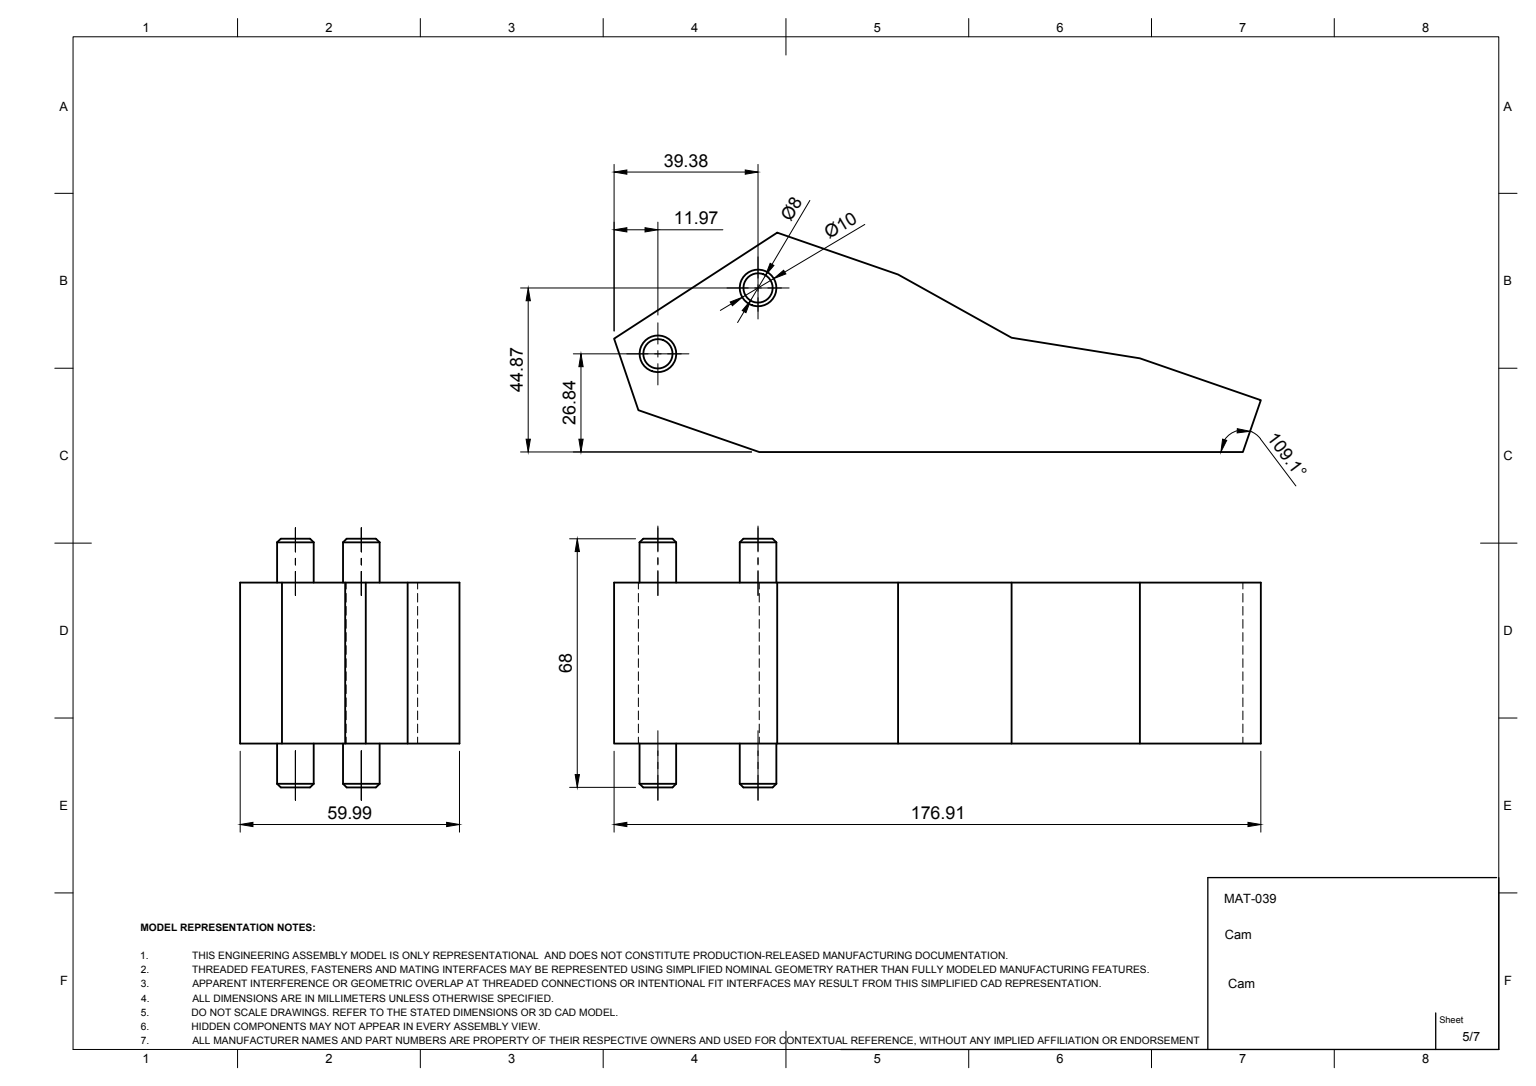
ISO-10303-21;
HEADER;
/* Generated by software containing ST-Developer
 * from STEP Tools, Inc. (www.steptools.com) 
 */

FILE_DESCRIPTION(
/* description */ ('STEP AP214'),
/* implementation_level */ '2;1');

FILE_NAME(
/* name */ 'Cam.step',
/* time_stamp */ '2026-11-14T21:46:24-08:00',
/* author */ (''),
/* organization */ (''),
/* preprocessor_version */ 'ST-DEVELOPER v20.2',
/* originating_system */ 'Autodesk Translation Framework v15.17.0.0',
/* authorisation */ '');

FILE_SCHEMA (('AUTOMOTIVE_DESIGN { 1 0 10303 214 3 1 1 }'));
ENDSEC;

DATA;
#10=MECHANICAL_DESIGN_GEOMETRIC_PRESENTATION_REPRESENTATION('',(#95),#7783);
#81=SHAPE_REPRESENTATION_RELATIONSHIP('SRR','None',#7826,#88);
#88=ADVANCED_BREP_SHAPE_REPRESENTATION('',(#102),#7782);
#95=STYLED_ITEM('',(#7871),#102);
#102=MANIFOLD_SOLID_BREP('Body1',#4170);
#108=CONICAL_SURFACE('',#4664,5.,0.785398163397445);
#109=CONICAL_SURFACE('',#4668,5.,0.785398163397445);
#110=CONICAL_SURFACE('',#4672,3.99999999999998,0.785398163397453);
#111=CONICAL_SURFACE('',#4675,3.99999999999998,0.785398163397453);
#155=FACE_BOUND('',#1601,.T.);
#156=FACE_BOUND('',#1602,.T.);
#157=FACE_BOUND('',#1604,.T.);
#158=FACE_BOUND('',#1605,.T.);
#274=PLANE('',#4686);
#275=PLANE('',#4687);
#276=PLANE('',#4688);
#277=PLANE('',#4689);
#278=PLANE('',#4690);
#279=PLANE('',#4691);
#280=PLANE('',#4692);
#281=PLANE('',#4693);
#282=PLANE('',#4694);
#283=PLANE('',#4695);
#284=PLANE('',#4696);
#285=PLANE('',#4697);
#286=PLANE('',#4698);
#287=PLANE('',#4699);
#288=PLANE('',#4700);
#613=LINE('',#7655,#972);
#614=LINE('',#7663,#973);
#615=LINE('',#7669,#974);
#616=LINE('',#7675,#975);
#617=LINE('',#7680,#976);
#618=LINE('',#7683,#977);
#619=LINE('',#7688,#978);
#620=LINE('',#7691,#979);
#621=LINE('',#7696,#980);
#622=LINE('',#7698,#981);
#623=LINE('',#7700,#982);
#624=LINE('',#7702,#983);
#625=LINE('',#7704,#984);
#626=LINE('',#7706,#985);
#627=LINE('',#7708,#986);
#628=LINE('',#7710,#987);
#629=LINE('',#7711,#988);
#630=LINE('',#7715,#989);
#631=LINE('',#7717,#990);
#632=LINE('',#7719,#991);
#633=LINE('',#7721,#992);
#634=LINE('',#7723,#993);
#635=LINE('',#7725,#994);
#636=LINE('',#7727,#995);
#637=LINE('',#7729,#996);
#638=LINE('',#7730,#997);
#639=LINE('',#7732,#998);
#640=LINE('',#7733,#999);
#641=LINE('',#7735,#1000);
#642=LINE('',#7737,#1001);
#643=LINE('',#7739,#1002);
#644=LINE('',#7741,#1003);
#645=LINE('',#7743,#1004);
#646=LINE('',#7745,#1005);
#647=LINE('',#7747,#1006);
#972=VECTOR('',#5872,5.);
#973=VECTOR('',#5881,5.);
#974=VECTOR('',#5888,3.99999999999998);
#975=VECTOR('',#5895,3.99999999999998);
#976=VECTOR('',#5902,5.);
#977=VECTOR('',#5905,5.);
#978=VECTOR('',#5912,5.);
#979=VECTOR('',#5915,5.);
#980=VECTOR('',#5920,1000.);
#981=VECTOR('',#5921,1000.);
#982=VECTOR('',#5922,1000.);
#983=VECTOR('',#5923,1000.);
#984=VECTOR('',#5924,1000.);
#985=VECTOR('',#5925,1000.);
#986=VECTOR('',#5926,1000.);
#987=VECTOR('',#5927,1000.);
#988=VECTOR('',#5928,1000.);
#989=VECTOR('',#5931,1000.);
#990=VECTOR('',#5932,1000.);
#991=VECTOR('',#5933,1000.);
#992=VECTOR('',#5934,1000.);
#993=VECTOR('',#5935,1000.);
#994=VECTOR('',#5936,1000.);
#995=VECTOR('',#5937,1000.);
#996=VECTOR('',#5938,1000.);
#997=VECTOR('',#5939,1000.);
#998=VECTOR('',#5942,1000.);
#999=VECTOR('',#5943,1000.);
#1000=VECTOR('',#5946,1000.);
#1001=VECTOR('',#5949,1000.);
#1002=VECTOR('',#5952,1000.);
#1003=VECTOR('',#5955,1000.);
#1004=VECTOR('',#5958,1000.);
#1005=VECTOR('',#5961,1000.);
#1006=VECTOR('',#5964,1000.);
#1082=CYLINDRICAL_SURFACE('',#4678,5.);
#1083=CYLINDRICAL_SURFACE('',#4680,5.);
#1084=CYLINDRICAL_SURFACE('',#4682,5.);
#1085=CYLINDRICAL_SURFACE('',#4684,5.);
#1306=FACE_OUTER_BOUND('',#1592,.T.);
#1307=FACE_OUTER_BOUND('',#1593,.T.);
#1308=FACE_OUTER_BOUND('',#1594,.T.);
#1309=FACE_OUTER_BOUND('',#1595,.T.);
#1310=FACE_OUTER_BOUND('',#1596,.T.);
#1311=FACE_OUTER_BOUND('',#1597,.T.);
#1312=FACE_OUTER_BOUND('',#1598,.T.);
#1313=FACE_OUTER_BOUND('',#1599,.T.);
#1314=FACE_OUTER_BOUND('',#1600,.T.);
#1315=FACE_OUTER_BOUND('',#1603,.T.);
#1316=FACE_OUTER_BOUND('',#1606,.T.);
#1317=FACE_OUTER_BOUND('',#1607,.T.);
#1318=FACE_OUTER_BOUND('',#1608,.T.);
#1319=FACE_OUTER_BOUND('',#1609,.T.);
#1320=FACE_OUTER_BOUND('',#1610,.T.);
#1321=FACE_OUTER_BOUND('',#1611,.T.);
#1322=FACE_OUTER_BOUND('',#1612,.T.);
#1323=FACE_OUTER_BOUND('',#1613,.T.);
#1324=FACE_OUTER_BOUND('',#1614,.T.);
#1325=FACE_OUTER_BOUND('',#1615,.T.);
#1326=FACE_OUTER_BOUND('',#1616,.T.);
#1327=FACE_OUTER_BOUND('',#1617,.T.);
#1328=FACE_OUTER_BOUND('',#1618,.T.);
#1592=EDGE_LOOP('',(#3804,#3805,#3806,#3807,#3808));
#1593=EDGE_LOOP('',(#3809,#3810,#3811,#3812,#3813));
#1594=EDGE_LOOP('',(#3814,#3815,#3816,#3817));
#1595=EDGE_LOOP('',(#3818,#3819,#3820,#3821));
#1596=EDGE_LOOP('',(#3822,#3823,#3824,#3825));
#1597=EDGE_LOOP('',(#3826,#3827,#3828,#3829,#3830));
#1598=EDGE_LOOP('',(#3831,#3832,#3833,#3834));
#1599=EDGE_LOOP('',(#3835,#3836,#3837,#3838,#3839));
#1600=EDGE_LOOP('',(#3840,#3841,#3842,#3843,#3844,#3845,#3846,#3847,#3848));
#1601=EDGE_LOOP('',(#3849));
#1602=EDGE_LOOP('',(#3850));
#1603=EDGE_LOOP('',(#3851,#3852,#3853,#3854,#3855,#3856,#3857,#3858,#3859));
#1604=EDGE_LOOP('',(#3860));
#1605=EDGE_LOOP('',(#3861));
#1606=EDGE_LOOP('',(#3862,#3863,#3864,#3865));
#1607=EDGE_LOOP('',(#3866,#3867,#3868,#3869));
#1608=EDGE_LOOP('',(#3870,#3871,#3872,#3873));
#1609=EDGE_LOOP('',(#3874,#3875,#3876,#3877));
#1610=EDGE_LOOP('',(#3878,#3879,#3880,#3881));
#1611=EDGE_LOOP('',(#3882,#3883,#3884,#3885));
#1612=EDGE_LOOP('',(#3886,#3887,#3888,#3889));
#1613=EDGE_LOOP('',(#3890,#3891,#3892,#3893));
#1614=EDGE_LOOP('',(#3894,#3895,#3896,#3897));
#1615=EDGE_LOOP('',(#3898));
#1616=EDGE_LOOP('',(#3899));
#1617=EDGE_LOOP('',(#3900));
#1618=EDGE_LOOP('',(#3901));
#1808=CIRCLE('',#4665,5.);
#1809=CIRCLE('',#4666,5.);
#1810=CIRCLE('',#4667,3.99999999999999);
#1811=CIRCLE('',#4669,5.);
#1812=CIRCLE('',#4670,5.);
#1813=CIRCLE('',#4671,3.99999999999999);
#1814=CIRCLE('',#4673,5.);
#1815=CIRCLE('',#4674,3.99999999999998);
#1816=CIRCLE('',#4676,5.);
#1817=CIRCLE('',#4677,3.99999999999998);
#1818=CIRCLE('',#4679,5.);
#1819=CIRCLE('',#4681,5.);
#1820=CIRCLE('',#4683,5.);
#1821=CIRCLE('',#4685,5.);
#2154=VERTEX_POINT('',#7650);
#2155=VERTEX_POINT('',#7651);
#2156=VERTEX_POINT('',#7654);
#2157=VERTEX_POINT('',#7658);
#2158=VERTEX_POINT('',#7659);
#2159=VERTEX_POINT('',#7662);
#2160=VERTEX_POINT('',#7666);
#2161=VERTEX_POINT('',#7668);
#2162=VERTEX_POINT('',#7672);
#2163=VERTEX_POINT('',#7674);
#2164=VERTEX_POINT('',#7678);
#2165=VERTEX_POINT('',#7682);
#2166=VERTEX_POINT('',#7686);
#2167=VERTEX_POINT('',#7690);
#2168=VERTEX_POINT('',#7694);
#2169=VERTEX_POINT('',#7695);
#2170=VERTEX_POINT('',#7697);
#2171=VERTEX_POINT('',#7699);
#2172=VERTEX_POINT('',#7701);
#2173=VERTEX_POINT('',#7703);
#2174=VERTEX_POINT('',#7705);
#2175=VERTEX_POINT('',#7707);
#2176=VERTEX_POINT('',#7709);
#2177=VERTEX_POINT('',#7713);
#2178=VERTEX_POINT('',#7714);
#2179=VERTEX_POINT('',#7716);
#2180=VERTEX_POINT('',#7718);
#2181=VERTEX_POINT('',#7720);
#2182=VERTEX_POINT('',#7722);
#2183=VERTEX_POINT('',#7724);
#2184=VERTEX_POINT('',#7726);
#2185=VERTEX_POINT('',#7728);
#2709=EDGE_CURVE('',#2154,#2155,#1808,.T.);
#2710=EDGE_CURVE('',#2155,#2154,#1809,.T.);
#2711=EDGE_CURVE('',#2155,#2156,#613,.T.);
#2712=EDGE_CURVE('',#2156,#2156,#1810,.T.);
#2713=EDGE_CURVE('',#2157,#2158,#1811,.T.);
#2714=EDGE_CURVE('',#2158,#2157,#1812,.T.);
#2715=EDGE_CURVE('',#2158,#2159,#614,.T.);
#2716=EDGE_CURVE('',#2159,#2159,#1813,.T.);
#2717=EDGE_CURVE('',#2160,#2160,#1814,.T.);
#2718=EDGE_CURVE('',#2160,#2161,#615,.T.);
#2719=EDGE_CURVE('',#2161,#2161,#1815,.T.);
#2720=EDGE_CURVE('',#2162,#2162,#1816,.T.);
#2721=EDGE_CURVE('',#2162,#2163,#616,.T.);
#2722=EDGE_CURVE('',#2163,#2163,#1817,.T.);
#2723=EDGE_CURVE('',#2164,#2164,#1818,.T.);
#2724=EDGE_CURVE('',#2164,#2162,#617,.T.);
#2725=EDGE_CURVE('',#2157,#2165,#618,.T.);
#2726=EDGE_CURVE('',#2165,#2165,#1819,.T.);
#2727=EDGE_CURVE('',#2166,#2166,#1820,.T.);
#2728=EDGE_CURVE('',#2166,#2160,#619,.T.);
#2729=EDGE_CURVE('',#2154,#2167,#620,.T.);
#2730=EDGE_CURVE('',#2167,#2167,#1821,.T.);
#2731=EDGE_CURVE('',#2168,#2169,#621,.T.);
#2732=EDGE_CURVE('',#2169,#2170,#622,.T.);
#2733=EDGE_CURVE('',#2170,#2171,#623,.T.);
#2734=EDGE_CURVE('',#2171,#2172,#624,.T.);
#2735=EDGE_CURVE('',#2172,#2173,#625,.T.);
#2736=EDGE_CURVE('',#2173,#2174,#626,.T.);
#2737=EDGE_CURVE('',#2174,#2175,#627,.T.);
#2738=EDGE_CURVE('',#2175,#2176,#628,.T.);
#2739=EDGE_CURVE('',#2176,#2168,#629,.T.);
#2740=EDGE_CURVE('',#2177,#2178,#630,.T.);
#2741=EDGE_CURVE('',#2179,#2177,#631,.T.);
#2742=EDGE_CURVE('',#2180,#2179,#632,.T.);
#2743=EDGE_CURVE('',#2181,#2180,#633,.T.);
#2744=EDGE_CURVE('',#2182,#2181,#634,.T.);
#2745=EDGE_CURVE('',#2183,#2182,#635,.T.);
#2746=EDGE_CURVE('',#2184,#2183,#636,.T.);
#2747=EDGE_CURVE('',#2185,#2184,#637,.T.);
#2748=EDGE_CURVE('',#2178,#2185,#638,.T.);
#2749=EDGE_CURVE('',#2169,#2178,#639,.T.);
#2750=EDGE_CURVE('',#2168,#2177,#640,.T.);
#2751=EDGE_CURVE('',#2170,#2185,#641,.T.);
#2752=EDGE_CURVE('',#2171,#2184,#642,.T.);
#2753=EDGE_CURVE('',#2172,#2183,#643,.T.);
#2754=EDGE_CURVE('',#2173,#2182,#644,.T.);
#2755=EDGE_CURVE('',#2174,#2181,#645,.T.);
#2756=EDGE_CURVE('',#2175,#2180,#646,.T.);
#2757=EDGE_CURVE('',#2176,#2179,#647,.T.);
#3804=ORIENTED_EDGE('',*,*,#2709,.F.);
#3805=ORIENTED_EDGE('',*,*,#2710,.F.);
#3806=ORIENTED_EDGE('',*,*,#2711,.T.);
#3807=ORIENTED_EDGE('',*,*,#2712,.F.);
#3808=ORIENTED_EDGE('',*,*,#2711,.F.);
#3809=ORIENTED_EDGE('',*,*,#2713,.F.);
#3810=ORIENTED_EDGE('',*,*,#2714,.F.);
#3811=ORIENTED_EDGE('',*,*,#2715,.T.);
#3812=ORIENTED_EDGE('',*,*,#2716,.F.);
#3813=ORIENTED_EDGE('',*,*,#2715,.F.);
#3814=ORIENTED_EDGE('',*,*,#2717,.F.);
#3815=ORIENTED_EDGE('',*,*,#2718,.T.);
#3816=ORIENTED_EDGE('',*,*,#2719,.F.);
#3817=ORIENTED_EDGE('',*,*,#2718,.F.);
#3818=ORIENTED_EDGE('',*,*,#2720,.F.);
#3819=ORIENTED_EDGE('',*,*,#2721,.T.);
#3820=ORIENTED_EDGE('',*,*,#2722,.F.);
#3821=ORIENTED_EDGE('',*,*,#2721,.F.);
#3822=ORIENTED_EDGE('',*,*,#2723,.T.);
#3823=ORIENTED_EDGE('',*,*,#2724,.T.);
#3824=ORIENTED_EDGE('',*,*,#2720,.T.);
#3825=ORIENTED_EDGE('',*,*,#2724,.F.);
#3826=ORIENTED_EDGE('',*,*,#2713,.T.);
#3827=ORIENTED_EDGE('',*,*,#2714,.T.);
#3828=ORIENTED_EDGE('',*,*,#2725,.T.);
#3829=ORIENTED_EDGE('',*,*,#2726,.T.);
#3830=ORIENTED_EDGE('',*,*,#2725,.F.);
#3831=ORIENTED_EDGE('',*,*,#2727,.T.);
#3832=ORIENTED_EDGE('',*,*,#2728,.T.);
#3833=ORIENTED_EDGE('',*,*,#2717,.T.);
#3834=ORIENTED_EDGE('',*,*,#2728,.F.);
#3835=ORIENTED_EDGE('',*,*,#2709,.T.);
#3836=ORIENTED_EDGE('',*,*,#2710,.T.);
#3837=ORIENTED_EDGE('',*,*,#2729,.T.);
#3838=ORIENTED_EDGE('',*,*,#2730,.T.);
#3839=ORIENTED_EDGE('',*,*,#2729,.F.);
#3840=ORIENTED_EDGE('',*,*,#2731,.T.);
#3841=ORIENTED_EDGE('',*,*,#2732,.T.);
#3842=ORIENTED_EDGE('',*,*,#2733,.T.);
#3843=ORIENTED_EDGE('',*,*,#2734,.T.);
#3844=ORIENTED_EDGE('',*,*,#2735,.T.);
#3845=ORIENTED_EDGE('',*,*,#2736,.T.);
#3846=ORIENTED_EDGE('',*,*,#2737,.T.);
#3847=ORIENTED_EDGE('',*,*,#2738,.T.);
#3848=ORIENTED_EDGE('',*,*,#2739,.T.);
#3849=ORIENTED_EDGE('',*,*,#2727,.F.);
#3850=ORIENTED_EDGE('',*,*,#2723,.F.);
#3851=ORIENTED_EDGE('',*,*,#2740,.F.);
#3852=ORIENTED_EDGE('',*,*,#2741,.F.);
#3853=ORIENTED_EDGE('',*,*,#2742,.F.);
#3854=ORIENTED_EDGE('',*,*,#2743,.F.);
#3855=ORIENTED_EDGE('',*,*,#2744,.F.);
#3856=ORIENTED_EDGE('',*,*,#2745,.F.);
#3857=ORIENTED_EDGE('',*,*,#2746,.F.);
#3858=ORIENTED_EDGE('',*,*,#2747,.F.);
#3859=ORIENTED_EDGE('',*,*,#2748,.F.);
#3860=ORIENTED_EDGE('',*,*,#2730,.F.);
#3861=ORIENTED_EDGE('',*,*,#2726,.F.);
#3862=ORIENTED_EDGE('',*,*,#2740,.T.);
#3863=ORIENTED_EDGE('',*,*,#2749,.F.);
#3864=ORIENTED_EDGE('',*,*,#2731,.F.);
#3865=ORIENTED_EDGE('',*,*,#2750,.T.);
#3866=ORIENTED_EDGE('',*,*,#2748,.T.);
#3867=ORIENTED_EDGE('',*,*,#2751,.F.);
#3868=ORIENTED_EDGE('',*,*,#2732,.F.);
#3869=ORIENTED_EDGE('',*,*,#2749,.T.);
#3870=ORIENTED_EDGE('',*,*,#2747,.T.);
#3871=ORIENTED_EDGE('',*,*,#2752,.F.);
#3872=ORIENTED_EDGE('',*,*,#2733,.F.);
#3873=ORIENTED_EDGE('',*,*,#2751,.T.);
#3874=ORIENTED_EDGE('',*,*,#2746,.T.);
#3875=ORIENTED_EDGE('',*,*,#2753,.F.);
#3876=ORIENTED_EDGE('',*,*,#2734,.F.);
#3877=ORIENTED_EDGE('',*,*,#2752,.T.);
#3878=ORIENTED_EDGE('',*,*,#2745,.T.);
#3879=ORIENTED_EDGE('',*,*,#2754,.F.);
#3880=ORIENTED_EDGE('',*,*,#2735,.F.);
#3881=ORIENTED_EDGE('',*,*,#2753,.T.);
#3882=ORIENTED_EDGE('',*,*,#2744,.T.);
#3883=ORIENTED_EDGE('',*,*,#2755,.F.);
#3884=ORIENTED_EDGE('',*,*,#2736,.F.);
#3885=ORIENTED_EDGE('',*,*,#2754,.T.);
#3886=ORIENTED_EDGE('',*,*,#2743,.T.);
#3887=ORIENTED_EDGE('',*,*,#2756,.F.);
#3888=ORIENTED_EDGE('',*,*,#2737,.F.);
#3889=ORIENTED_EDGE('',*,*,#2755,.T.);
#3890=ORIENTED_EDGE('',*,*,#2742,.T.);
#3891=ORIENTED_EDGE('',*,*,#2757,.F.);
#3892=ORIENTED_EDGE('',*,*,#2738,.F.);
#3893=ORIENTED_EDGE('',*,*,#2756,.T.);
#3894=ORIENTED_EDGE('',*,*,#2741,.T.);
#3895=ORIENTED_EDGE('',*,*,#2750,.F.);
#3896=ORIENTED_EDGE('',*,*,#2739,.F.);
#3897=ORIENTED_EDGE('',*,*,#2757,.T.);
#3898=ORIENTED_EDGE('',*,*,#2712,.T.);
#3899=ORIENTED_EDGE('',*,*,#2719,.T.);
#3900=ORIENTED_EDGE('',*,*,#2716,.T.);
#3901=ORIENTED_EDGE('',*,*,#2722,.T.);
#4141=ADVANCED_FACE('',(#1306),#108,.T.);
#4142=ADVANCED_FACE('',(#1307),#109,.T.);
#4143=ADVANCED_FACE('',(#1308),#110,.T.);
#4144=ADVANCED_FACE('',(#1309),#111,.T.);
#4145=ADVANCED_FACE('',(#1310),#1082,.T.);
#4146=ADVANCED_FACE('',(#1311),#1083,.T.);
#4147=ADVANCED_FACE('',(#1312),#1084,.T.);
#4148=ADVANCED_FACE('',(#1313),#1085,.T.);
#4149=ADVANCED_FACE('',(#1314,#155,#156),#274,.T.);
#4150=ADVANCED_FACE('',(#1315,#157,#158),#275,.F.);
#4151=ADVANCED_FACE('',(#1316),#276,.F.);
#4152=ADVANCED_FACE('',(#1317),#277,.F.);
#4153=ADVANCED_FACE('',(#1318),#278,.F.);
#4154=ADVANCED_FACE('',(#1319),#279,.F.);
#4155=ADVANCED_FACE('',(#1320),#280,.F.);
#4156=ADVANCED_FACE('',(#1321),#281,.F.);
#4157=ADVANCED_FACE('',(#1322),#282,.F.);
#4158=ADVANCED_FACE('',(#1323),#283,.F.);
#4159=ADVANCED_FACE('',(#1324),#284,.F.);
#4160=ADVANCED_FACE('',(#1325),#285,.F.);
#4161=ADVANCED_FACE('',(#1326),#286,.T.);
#4162=ADVANCED_FACE('',(#1327),#287,.F.);
#4163=ADVANCED_FACE('',(#1328),#288,.T.);
#4170=CLOSED_SHELL('',(#4141,#4142,#4143,#4144,#4145,#4146,#4147,#4148,
#4149,#4150,#4151,#4152,#4153,#4154,#4155,#4156,#4157,#4158,#4159,#4160,
#4161,#4162,#4163));
#4663=AXIS2_PLACEMENT_3D('',#7648,#5864,#5865);
#4664=AXIS2_PLACEMENT_3D('',#7649,#5866,#5867);
#4665=AXIS2_PLACEMENT_3D('',#7652,#5868,#5869);
#4666=AXIS2_PLACEMENT_3D('',#7653,#5870,#5871);
#4667=AXIS2_PLACEMENT_3D('',#7656,#5873,#5874);
#4668=AXIS2_PLACEMENT_3D('',#7657,#5875,#5876);
#4669=AXIS2_PLACEMENT_3D('',#7660,#5877,#5878);
#4670=AXIS2_PLACEMENT_3D('',#7661,#5879,#5880);
#4671=AXIS2_PLACEMENT_3D('',#7664,#5882,#5883);
#4672=AXIS2_PLACEMENT_3D('',#7665,#5884,#5885);
#4673=AXIS2_PLACEMENT_3D('',#7667,#5886,#5887);
#4674=AXIS2_PLACEMENT_3D('',#7670,#5889,#5890);
#4675=AXIS2_PLACEMENT_3D('',#7671,#5891,#5892);
#4676=AXIS2_PLACEMENT_3D('',#7673,#5893,#5894);
#4677=AXIS2_PLACEMENT_3D('',#7676,#5896,#5897);
#4678=AXIS2_PLACEMENT_3D('',#7677,#5898,#5899);
#4679=AXIS2_PLACEMENT_3D('',#7679,#5900,#5901);
#4680=AXIS2_PLACEMENT_3D('',#7681,#5903,#5904);
#4681=AXIS2_PLACEMENT_3D('',#7684,#5906,#5907);
#4682=AXIS2_PLACEMENT_3D('',#7685,#5908,#5909);
#4683=AXIS2_PLACEMENT_3D('',#7687,#5910,#5911);
#4684=AXIS2_PLACEMENT_3D('',#7689,#5913,#5914);
#4685=AXIS2_PLACEMENT_3D('',#7692,#5916,#5917);
#4686=AXIS2_PLACEMENT_3D('',#7693,#5918,#5919);
#4687=AXIS2_PLACEMENT_3D('',#7712,#5929,#5930);
#4688=AXIS2_PLACEMENT_3D('',#7731,#5940,#5941);
#4689=AXIS2_PLACEMENT_3D('',#7734,#5944,#5945);
#4690=AXIS2_PLACEMENT_3D('',#7736,#5947,#5948);
#4691=AXIS2_PLACEMENT_3D('',#7738,#5950,#5951);
#4692=AXIS2_PLACEMENT_3D('',#7740,#5953,#5954);
#4693=AXIS2_PLACEMENT_3D('',#7742,#5956,#5957);
#4694=AXIS2_PLACEMENT_3D('',#7744,#5959,#5960);
#4695=AXIS2_PLACEMENT_3D('',#7746,#5962,#5963);
#4696=AXIS2_PLACEMENT_3D('',#7748,#5965,#5966);
#4697=AXIS2_PLACEMENT_3D('',#7749,#5967,#5968);
#4698=AXIS2_PLACEMENT_3D('',#7750,#5969,#5970);
#4699=AXIS2_PLACEMENT_3D('',#7751,#5971,#5972);
#4700=AXIS2_PLACEMENT_3D('',#7752,#5973,#5974);
#5864=DIRECTION('axis',(0.,0.,1.));
#5865=DIRECTION('refdir',(1.,0.,0.));
#5866=DIRECTION('center_axis',(0.,0.,1.));
#5867=DIRECTION('ref_axis',(1.,0.,0.));
#5868=DIRECTION('center_axis',(0.,0.,1.));
#5869=DIRECTION('ref_axis',(1.,0.,0.));
#5870=DIRECTION('center_axis',(0.,0.,1.));
#5871=DIRECTION('ref_axis',(1.,0.,0.));
#5872=DIRECTION('',(0.707106781186545,8.6595605623549E-17,-0.70710678118655));
#5873=DIRECTION('center_axis',(0.,0.,-1.));
#5874=DIRECTION('ref_axis',(1.,0.,0.));
#5875=DIRECTION('center_axis',(0.,0.,1.));
#5876=DIRECTION('ref_axis',(1.,0.,0.));
#5877=DIRECTION('center_axis',(0.,0.,1.));
#5878=DIRECTION('ref_axis',(1.,0.,0.));
#5879=DIRECTION('center_axis',(0.,0.,1.));
#5880=DIRECTION('ref_axis',(1.,0.,0.));
#5881=DIRECTION('',(0.707106781186545,8.6595605623549E-17,-0.70710678118655));
#5882=DIRECTION('center_axis',(0.,0.,-1.));
#5883=DIRECTION('ref_axis',(1.,0.,0.));
#5884=DIRECTION('center_axis',(0.,0.,-1.));
#5885=DIRECTION('ref_axis',(-1.,0.,0.));
#5886=DIRECTION('center_axis',(0.,0.,-1.));
#5887=DIRECTION('ref_axis',(1.,0.,0.));
#5888=DIRECTION('',(-0.707106781186551,8.65956056235498E-17,0.707106781186544));
#5889=DIRECTION('center_axis',(0.,0.,1.));
#5890=DIRECTION('ref_axis',(1.,0.,0.));
#5891=DIRECTION('center_axis',(0.,0.,-1.));
#5892=DIRECTION('ref_axis',(-1.,0.,0.));
#5893=DIRECTION('center_axis',(0.,0.,-1.));
#5894=DIRECTION('ref_axis',(1.,0.,0.));
#5895=DIRECTION('',(-0.707106781186551,8.65956056235497E-17,0.707106781186544));
#5896=DIRECTION('center_axis',(0.,0.,1.));
#5897=DIRECTION('ref_axis',(1.,0.,0.));
#5898=DIRECTION('center_axis',(0.,0.,-1.));
#5899=DIRECTION('ref_axis',(-1.,0.,0.));
#5900=DIRECTION('center_axis',(0.,0.,1.));
#5901=DIRECTION('ref_axis',(1.,0.,0.));
#5902=DIRECTION('',(0.,0.,1.));
#5903=DIRECTION('center_axis',(0.,0.,-1.));
#5904=DIRECTION('ref_axis',(-1.,0.,0.));
#5905=DIRECTION('',(0.,0.,1.));
#5906=DIRECTION('center_axis',(0.,0.,-1.));
#5907=DIRECTION('ref_axis',(1.,0.,0.));
#5908=DIRECTION('center_axis',(0.,0.,-1.));
#5909=DIRECTION('ref_axis',(-1.,0.,0.));
#5910=DIRECTION('center_axis',(0.,0.,1.));
#5911=DIRECTION('ref_axis',(1.,0.,0.));
#5912=DIRECTION('',(0.,0.,1.));
#5913=DIRECTION('center_axis',(0.,0.,-1.));
#5914=DIRECTION('ref_axis',(-1.,0.,0.));
#5915=DIRECTION('',(0.,0.,1.));
#5916=DIRECTION('center_axis',(0.,0.,-1.));
#5917=DIRECTION('ref_axis',(1.,0.,0.));
#5918=DIRECTION('center_axis',(0.,0.,1.));
#5919=DIRECTION('ref_axis',(1.,0.,0.));
#5920=DIRECTION('',(-0.613967345345676,-0.789331425225921,0.));
#5921=DIRECTION('',(0.613967345345676,-0.78933142522592,0.));
#5922=DIRECTION('',(1.,1.98254111540207E-16,0.));
#5923=DIRECTION('',(0.984807753012208,0.173648177666931,0.));
#5924=DIRECTION('',(0.984807753012208,-0.173648177666931,0.));
#5925=DIRECTION('',(1.,0.,0.));
#5926=DIRECTION('',(0.,1.,0.));
#5927=DIRECTION('',(-0.944943348295466,0.327233966012321,0.));
#5928=DIRECTION('',(-1.,1.98254111540207E-16,0.));
#5929=DIRECTION('center_axis',(0.,0.,1.));
#5930=DIRECTION('ref_axis',(1.,0.,0.));
#5931=DIRECTION('',(-0.613967345345676,-0.789331425225921,0.));
#5932=DIRECTION('',(-1.,1.98254111540207E-16,0.));
#5933=DIRECTION('',(-0.944943348295466,0.327233966012321,0.));
#5934=DIRECTION('',(0.,1.,0.));
#5935=DIRECTION('',(1.,0.,0.));
#5936=DIRECTION('',(0.984807753012208,-0.173648177666931,0.));
#5937=DIRECTION('',(0.984807753012208,0.173648177666931,0.));
#5938=DIRECTION('',(1.,1.98254111540207E-16,0.));
#5939=DIRECTION('',(0.613967345345676,-0.78933142522592,0.));
#5940=DIRECTION('center_axis',(0.789331425225921,-0.613967345345676,0.));
#5941=DIRECTION('ref_axis',(0.613967345345676,0.789331425225921,0.));
#5942=DIRECTION('',(0.,0.,-1.));
#5943=DIRECTION('',(0.,0.,-1.));
#5944=DIRECTION('center_axis',(0.78933142522592,0.613967345345677,0.));
#5945=DIRECTION('ref_axis',(-0.613967345345677,0.78933142522592,0.));
#5946=DIRECTION('',(0.,0.,-1.));
#5947=DIRECTION('center_axis',(-1.98254111540206E-16,1.,0.));
#5948=DIRECTION('ref_axis',(-1.,-1.98254111540207E-16,0.));
#5949=DIRECTION('',(0.,0.,-1.));
#5950=DIRECTION('center_axis',(-0.173648177666931,0.984807753012208,0.));
#5951=DIRECTION('ref_axis',(-0.984807753012208,-0.173648177666931,0.));
#5952=DIRECTION('',(0.,0.,-1.));
#5953=DIRECTION('center_axis',(0.173648177666931,0.984807753012208,0.));
#5954=DIRECTION('ref_axis',(-0.984807753012208,0.173648177666931,0.));
#5955=DIRECTION('',(0.,0.,-1.));
#5956=DIRECTION('center_axis',(0.,1.,0.));
#5957=DIRECTION('ref_axis',(0.,0.,1.));
#5958=DIRECTION('',(0.,0.,-1.));
#5959=DIRECTION('center_axis',(-1.,0.,0.));
#5960=DIRECTION('ref_axis',(0.,0.,1.));
#5961=DIRECTION('',(0.,0.,-1.));
#5962=DIRECTION('center_axis',(-0.327233966012321,-0.944943348295466,0.));
#5963=DIRECTION('ref_axis',(0.944943348295467,-0.327233966012321,0.));
#5964=DIRECTION('',(0.,0.,-1.));
#5965=DIRECTION('center_axis',(-1.98254111540206E-16,-1.,0.));
#5966=DIRECTION('ref_axis',(1.,-1.98254111540207E-16,0.));
#5967=DIRECTION('center_axis',(0.,0.,1.));
#5968=DIRECTION('ref_axis',(1.,0.,0.));
#5969=DIRECTION('center_axis',(0.,0.,1.));
#5970=DIRECTION('ref_axis',(1.,0.,0.));
#5971=DIRECTION('center_axis',(0.,0.,1.));
#5972=DIRECTION('ref_axis',(1.,0.,0.));
#5973=DIRECTION('center_axis',(0.,0.,1.));
#5974=DIRECTION('ref_axis',(1.,0.,0.));
#7648=CARTESIAN_POINT('',(0.,0.,0.));
#7649=CARTESIAN_POINT('Origin',(20.,-26.,-33.));
#7650=CARTESIAN_POINT('',(25.,-26.,-33.));
#7651=CARTESIAN_POINT('',(15.,-26.,-33.));
#7652=CARTESIAN_POINT('Origin',(20.,-26.,-33.));
#7653=CARTESIAN_POINT('Origin',(20.,-26.,-33.));
#7654=CARTESIAN_POINT('',(16.,-26.,-34.));
#7655=CARTESIAN_POINT('',(15.,-26.,-33.));
#7656=CARTESIAN_POINT('Origin',(20.,-26.,-34.));
#7657=CARTESIAN_POINT('Origin',(0.,0.,-33.));
#7658=CARTESIAN_POINT('',(5.,6.12323399573677E-16,-33.));
#7659=CARTESIAN_POINT('',(-5.,-6.12323399573677E-16,-33.));
#7660=CARTESIAN_POINT('Origin',(0.,0.,-33.));
#7661=CARTESIAN_POINT('Origin',(0.,0.,-33.));
#7662=CARTESIAN_POINT('',(-3.99999999999999,-4.8985871965894E-16,-34.));
#7663=CARTESIAN_POINT('',(-5.,-6.12323399573677E-16,-33.));
#7664=CARTESIAN_POINT('Origin',(0.,0.,-34.));
#7665=CARTESIAN_POINT('Origin',(20.,-26.,34.));
#7666=CARTESIAN_POINT('',(25.,-26.,33.));
#7667=CARTESIAN_POINT('Origin',(20.,-26.,33.));
#7668=CARTESIAN_POINT('',(24.,-26.,34.));
#7669=CARTESIAN_POINT('',(24.,-26.,34.));
#7670=CARTESIAN_POINT('Origin',(20.,-26.,34.));
#7671=CARTESIAN_POINT('Origin',(0.,0.,34.));
#7672=CARTESIAN_POINT('',(5.,-6.12323399573677E-16,33.));
#7673=CARTESIAN_POINT('Origin',(0.,0.,33.));
#7674=CARTESIAN_POINT('',(3.99999999999998,-4.89858719658939E-16,34.));
#7675=CARTESIAN_POINT('',(3.99999999999998,-4.89858719658939E-16,34.));
#7676=CARTESIAN_POINT('Origin',(0.,0.,34.));
#7677=CARTESIAN_POINT('Origin',(0.,0.,34.));
#7678=CARTESIAN_POINT('',(5.,-6.12323399573677E-16,22.));
#7679=CARTESIAN_POINT('Origin',(0.,0.,22.));
#7680=CARTESIAN_POINT('',(5.,-6.12323399573677E-16,34.));
#7681=CARTESIAN_POINT('Origin',(0.,0.,34.));
#7682=CARTESIAN_POINT('',(5.,-6.12323399573677E-16,-22.));
#7683=CARTESIAN_POINT('',(5.,-6.12323399573677E-16,34.));
#7684=CARTESIAN_POINT('Origin',(0.,0.,-22.));
#7685=CARTESIAN_POINT('Origin',(20.,-26.,34.));
#7686=CARTESIAN_POINT('',(25.,-26.,22.));
#7687=CARTESIAN_POINT('Origin',(20.,-26.,22.));
#7688=CARTESIAN_POINT('',(25.,-26.,34.));
#7689=CARTESIAN_POINT('Origin',(20.,-26.,34.));
#7690=CARTESIAN_POINT('',(25.,-26.,-22.));
#7691=CARTESIAN_POINT('',(25.,-26.,34.));
#7692=CARTESIAN_POINT('Origin',(20.,-26.,-22.));
#7693=CARTESIAN_POINT('Origin',(-12.6689495444044,0.,22.));
#7694=CARTESIAN_POINT('',(1.26419667377704E-16,16.2875111776015,22.));
#7695=CARTESIAN_POINT('',(-12.6689495444044,2.44580763519679E-16,22.));
#7696=CARTESIAN_POINT('',(-12.6689495444044,2.44580763519679E-16,22.));
#7697=CARTESIAN_POINT('',(20.,-42.,22.));
#7698=CARTESIAN_POINT('',(20.,-42.,22.));
#7699=CARTESIAN_POINT('',(55.,-42.,22.));
#7700=CARTESIAN_POINT('',(55.,-42.,22.));
#7701=CARTESIAN_POINT('',(90.,-35.8285556752037,22.));
#7702=CARTESIAN_POINT('',(90.,-35.8285556752037,22.));
#7703=CARTESIAN_POINT('',(125.,-42.,22.));
#7704=CARTESIAN_POINT('',(125.,-42.,22.));
#7705=CARTESIAN_POINT('',(160.,-42.,22.));
#7706=CARTESIAN_POINT('',(160.,-42.,22.));
#7707=CARTESIAN_POINT('',(160.,-27.,22.));
#7708=CARTESIAN_POINT('',(160.,-27.,22.));
#7709=CARTESIAN_POINT('',(35.,16.2875111776015,22.));
#7710=CARTESIAN_POINT('',(35.,16.2875111776015,22.));
#7711=CARTESIAN_POINT('',(1.26419667377704E-16,16.2875111776015,22.));
#7712=CARTESIAN_POINT('Origin',(-12.6689495444044,0.,-22.));
#7713=CARTESIAN_POINT('',(1.26419667377704E-16,16.2875111776015,-22.));
#7714=CARTESIAN_POINT('',(-12.6689495444044,2.44580763519679E-16,-22.));
#7715=CARTESIAN_POINT('',(-12.6689495444044,2.44580763519679E-16,-22.));
#7716=CARTESIAN_POINT('',(35.,16.2875111776015,-22.));
#7717=CARTESIAN_POINT('',(1.26419667377704E-16,16.2875111776015,-22.));
#7718=CARTESIAN_POINT('',(160.,-27.,-22.));
#7719=CARTESIAN_POINT('',(35.,16.2875111776015,-22.));
#7720=CARTESIAN_POINT('',(160.,-42.,-22.));
#7721=CARTESIAN_POINT('',(160.,-27.,-22.));
#7722=CARTESIAN_POINT('',(125.,-42.,-22.));
#7723=CARTESIAN_POINT('',(160.,-42.,-22.));
#7724=CARTESIAN_POINT('',(90.,-35.8285556752037,-22.));
#7725=CARTESIAN_POINT('',(125.,-42.,-22.));
#7726=CARTESIAN_POINT('',(55.,-42.,-22.));
#7727=CARTESIAN_POINT('',(90.,-35.8285556752037,-22.));
#7728=CARTESIAN_POINT('',(20.,-42.,-22.));
#7729=CARTESIAN_POINT('',(55.,-42.,-22.));
#7730=CARTESIAN_POINT('',(20.,-42.,-22.));
#7731=CARTESIAN_POINT('Origin',(-12.6689495444044,2.44580763519679E-16,
22.));
#7732=CARTESIAN_POINT('',(-12.6689495444044,2.44580763519679E-16,22.));
#7733=CARTESIAN_POINT('',(1.26419667377704E-16,16.2875111776015,22.));
#7734=CARTESIAN_POINT('Origin',(20.,-42.,22.));
#7735=CARTESIAN_POINT('',(20.,-42.,22.));
#7736=CARTESIAN_POINT('Origin',(55.,-42.,22.));
#7737=CARTESIAN_POINT('',(55.,-42.,22.));
#7738=CARTESIAN_POINT('Origin',(90.,-35.8285556752037,22.));
#7739=CARTESIAN_POINT('',(90.,-35.8285556752037,22.));
#7740=CARTESIAN_POINT('Origin',(125.,-42.,22.));
#7741=CARTESIAN_POINT('',(125.,-42.,22.));
#7742=CARTESIAN_POINT('Origin',(160.,-42.,22.));
#7743=CARTESIAN_POINT('',(160.,-42.,22.));
#7744=CARTESIAN_POINT('Origin',(160.,-27.,22.));
#7745=CARTESIAN_POINT('',(160.,-27.,22.));
#7746=CARTESIAN_POINT('Origin',(35.,16.2875111776015,22.));
#7747=CARTESIAN_POINT('',(35.,16.2875111776015,22.));
#7748=CARTESIAN_POINT('Origin',(1.26419667377704E-16,16.2875111776015,22.));
#7749=CARTESIAN_POINT('Origin',(20.,-26.,-34.));
#7750=CARTESIAN_POINT('Origin',(20.,-26.,34.));
#7751=CARTESIAN_POINT('Origin',(0.,0.,-34.));
#7752=CARTESIAN_POINT('Origin',(0.,0.,34.));
#7772=UNCERTAINTY_MEASURE_WITH_UNIT(LENGTH_MEASURE(0.01),#7784,
'DISTANCE_ACCURACY_VALUE',
'Maximum model space distance between geometric entities at asserted c
onnectivities');
#7773=UNCERTAINTY_MEASURE_WITH_UNIT(LENGTH_MEASURE(0.01),#7784,
'DISTANCE_ACCURACY_VALUE',
'Maximum model space distance between geometric entities at asserted c
onnectivities');
#7782=(
GEOMETRIC_REPRESENTATION_CONTEXT(3)
GLOBAL_UNCERTAINTY_ASSIGNED_CONTEXT((#7772))
GLOBAL_UNIT_ASSIGNED_CONTEXT((#7784,#7786,#7787))
REPRESENTATION_CONTEXT('','3D')
);
#7783=(
GEOMETRIC_REPRESENTATION_CONTEXT(3)
GLOBAL_UNCERTAINTY_ASSIGNED_CONTEXT((#7773))
GLOBAL_UNIT_ASSIGNED_CONTEXT((#7784,#7786,#7787))
REPRESENTATION_CONTEXT('','3D')
);
#7784=(
LENGTH_UNIT()
NAMED_UNIT(*)
SI_UNIT(.MILLI.,.METRE.)
);
#7786=(
NAMED_UNIT(*)
PLANE_ANGLE_UNIT()
SI_UNIT($,.RADIAN.)
);
#7787=(
NAMED_UNIT(*)
SI_UNIT($,.STERADIAN.)
SOLID_ANGLE_UNIT()
);
#7796=SHAPE_DEFINITION_REPRESENTATION(#7806,#7826);
#7806=PRODUCT_DEFINITION_SHAPE('',$,#7836);
#7826=SHAPE_REPRESENTATION('',(#4663),#7782);
#7827=PRODUCT_DEFINITION_CONTEXT('part definition',#7856,'design');
#7836=PRODUCT_DEFINITION('Cam','Cam',#7845,#7827);
#7845=PRODUCT_DEFINITION_FORMATION('',$,#7866);
#7856=APPLICATION_CONTEXT(
'Core Data for Automotive Mechanical Design Process');
#7857=PRODUCT_CONTEXT('part definition',#7856,'mechanical');
#7866=PRODUCT('Cam','Cam',$,(#7857));
#7871=PRESENTATION_STYLE_ASSIGNMENT((#7876));
#7876=SURFACE_STYLE_USAGE(.BOTH.,#7881);
#7881=SURFACE_SIDE_STYLE('',(#7886));
#7886=SURFACE_STYLE_FILL_AREA(#7891);
#7891=FILL_AREA_STYLE('Opaque(227,224,212)',(#7896));
#7896=FILL_AREA_STYLE_COLOUR('Opaque(227,224,212)',#7901);
#7901=COLOUR_RGB('Opaque(227,224,212)',0.890196078431372,0.87843137254902,
0.831372549019608);
ENDSEC;
END-ISO-10303-21;
